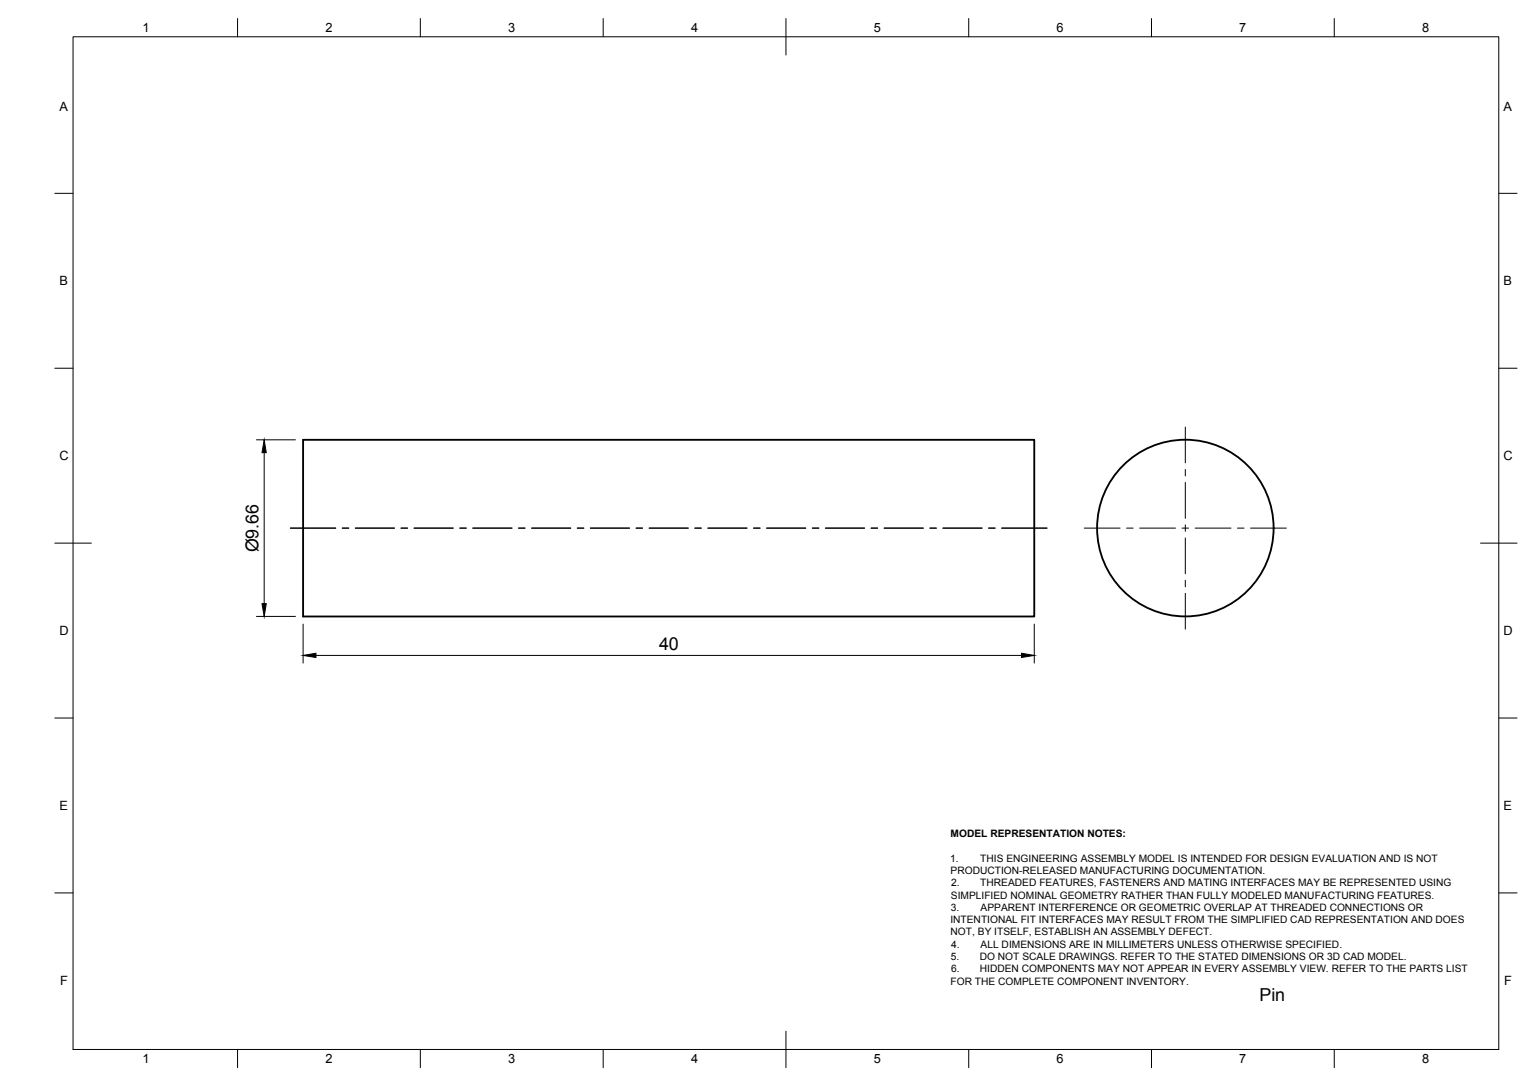
ISO-10303-21;
HEADER;
/* Generated by software containing ST-Developer
 * from STEP Tools, Inc. (www.steptools.com) 
 */

FILE_DESCRIPTION(
/* description */ ('STEP AP214'),
/* implementation_level */ '2;1');

FILE_NAME(
/* name */ 'PIN.step',
/* time_stamp */ '2026-10-06T11:20:11-07:00',
/* author */ (''),
/* organization */ (''),
/* preprocessor_version */ 'ST-DEVELOPER v20.2',
/* originating_system */ 'Autodesk Translation Framework v15.15.0.0',
/* authorisation */ '');

FILE_SCHEMA (('AUTOMOTIVE_DESIGN { 1 0 10303 214 3 1 1 }'));
ENDSEC;

DATA;
#10=MECHANICAL_DESIGN_GEOMETRIC_PRESENTATION_REPRESENTATION('',(#50),#2840);
#38=SHAPE_REPRESENTATION_RELATIONSHIP('SRR','None',#2869,#44);
#44=ADVANCED_BREP_SHAPE_REPRESENTATION('',(#56),#2837);
#50=STYLED_ITEM('',(#2905),#56);
#56=MANIFOLD_SOLID_BREP('Body1',#1550);
#109=PLANE('',#1747);
#110=PLANE('',#1748);
#175=FACE_OUTER_BOUND('',#290,.T.);
#176=FACE_OUTER_BOUND('',#291,.T.);
#177=FACE_OUTER_BOUND('',#292,.T.);
#290=EDGE_LOOP('',(#1202,#1203,#1204,#1205));
#291=EDGE_LOOP('',(#1206));
#292=EDGE_LOOP('',(#1207));
#373=LINE('',#2610,#466);
#466=VECTOR('',#2132,4.83000000000002);
#590=CIRCLE('',#1745,4.83000000000002);
#591=CIRCLE('',#1746,4.83000000000002);
#705=VERTEX_POINT('',#2607);
#706=VERTEX_POINT('',#2609);
#882=EDGE_CURVE('',#705,#705,#590,.T.);
#883=EDGE_CURVE('',#705,#706,#373,.T.);
#884=EDGE_CURVE('',#706,#706,#591,.T.);
#1202=ORIENTED_EDGE('',*,*,#882,.T.);
#1203=ORIENTED_EDGE('',*,*,#883,.T.);
#1204=ORIENTED_EDGE('',*,*,#884,.F.);
#1205=ORIENTED_EDGE('',*,*,#883,.F.);
#1206=ORIENTED_EDGE('',*,*,#884,.T.);
#1207=ORIENTED_EDGE('',*,*,#882,.F.);
#1433=CYLINDRICAL_SURFACE('',#1744,4.83000000000002);
#1506=ADVANCED_FACE('',(#175),#1433,.T.);
#1507=ADVANCED_FACE('',(#176),#109,.T.);
#1508=ADVANCED_FACE('',(#177),#110,.F.);
#1550=CLOSED_SHELL('',(#1506,#1507,#1508));
#1743=AXIS2_PLACEMENT_3D('',#2605,#2126,#2127);
#1744=AXIS2_PLACEMENT_3D('',#2606,#2128,#2129);
#1745=AXIS2_PLACEMENT_3D('',#2608,#2130,#2131);
#1746=AXIS2_PLACEMENT_3D('',#2611,#2133,#2134);
#1747=AXIS2_PLACEMENT_3D('',#2612,#2135,#2136);
#1748=AXIS2_PLACEMENT_3D('',#2613,#2137,#2138);
#2126=DIRECTION('axis',(0.,0.,1.));
#2127=DIRECTION('refdir',(1.,0.,0.));
#2128=DIRECTION('center_axis',(0.,-1.,0.));
#2129=DIRECTION('ref_axis',(-5.55111512312576E-17,0.,-1.));
#2130=DIRECTION('center_axis',(0.,1.,0.));
#2131=DIRECTION('ref_axis',(5.55111512312576E-17,0.,1.));
#2132=DIRECTION('',(0.,1.,0.));
#2133=DIRECTION('center_axis',(0.,1.,0.));
#2134=DIRECTION('ref_axis',(5.55111512312576E-17,0.,1.));
#2135=DIRECTION('center_axis',(0.,1.,0.));
#2136=DIRECTION('ref_axis',(5.55111512312576E-17,0.,1.));
#2137=DIRECTION('center_axis',(0.,1.,0.));
#2138=DIRECTION('ref_axis',(5.55111512312576E-17,0.,1.));
#2605=CARTESIAN_POINT('',(0.,0.,0.));
#2606=CARTESIAN_POINT('Origin',(0.,40.,0.));
#2607=CARTESIAN_POINT('',(-3.23385543541199E-16,0.,4.83000000000002));
#2608=CARTESIAN_POINT('Origin',(0.,0.,0.));
#2609=CARTESIAN_POINT('',(-3.23385543541199E-16,40.,4.83000000000002));
#2610=CARTESIAN_POINT('',(-3.23385543541199E-16,40.,4.83000000000002));
#2611=CARTESIAN_POINT('Origin',(0.,40.,0.));
#2612=CARTESIAN_POINT('Origin',(0.,40.,0.));
#2613=CARTESIAN_POINT('Origin',(0.,0.,0.));
#2829=UNCERTAINTY_MEASURE_WITH_UNIT(LENGTH_MEASURE(0.01),#2841,
'DISTANCE_ACCURACY_VALUE',
'Maximum model space distance between geometric entities at asserted c
onnectivities');
#2832=UNCERTAINTY_MEASURE_WITH_UNIT(LENGTH_MEASURE(0.01),#2841,
'DISTANCE_ACCURACY_VALUE',
'Maximum model space distance between geometric entities at asserted c
onnectivities');
#2837=(
GEOMETRIC_REPRESENTATION_CONTEXT(3)
GLOBAL_UNCERTAINTY_ASSIGNED_CONTEXT((#2829))
GLOBAL_UNIT_ASSIGNED_CONTEXT((#2841,#2843,#2844))
REPRESENTATION_CONTEXT('','3D')
);
#2840=(
GEOMETRIC_REPRESENTATION_CONTEXT(3)
GLOBAL_UNCERTAINTY_ASSIGNED_CONTEXT((#2832))
GLOBAL_UNIT_ASSIGNED_CONTEXT((#2841,#2843,#2844))
REPRESENTATION_CONTEXT('','3D')
);
#2841=(
LENGTH_UNIT()
NAMED_UNIT(*)
SI_UNIT(.MILLI.,.METRE.)
);
#2843=(
NAMED_UNIT(*)
PLANE_ANGLE_UNIT()
SI_UNIT($,.RADIAN.)
);
#2844=(
NAMED_UNIT(*)
SI_UNIT($,.STERADIAN.)
SOLID_ANGLE_UNIT()
);
#2849=SHAPE_DEFINITION_REPRESENTATION(#2856,#2869);
#2856=PRODUCT_DEFINITION_SHAPE('',$,#2877);
#2869=SHAPE_REPRESENTATION('',(#1743),#2837);
#2872=PRODUCT_DEFINITION_CONTEXT('part definition',#2895,'design');
#2877=PRODUCT_DEFINITION('Pin','PIN',#2884,#2872);
#2884=PRODUCT_DEFINITION_FORMATION('',$,#2901);
#2895=APPLICATION_CONTEXT(
'Core Data for Automotive Mechanical Design Process');
#2896=PRODUCT_CONTEXT('part definition',#2895,'mechanical');
#2901=PRODUCT('Pin','PIN',$,(#2896));
#2905=PRESENTATION_STYLE_ASSIGNMENT((#2907));
#2907=SURFACE_STYLE_USAGE(.BOTH.,#2909);
#2909=SURFACE_SIDE_STYLE('',(#2911));
#2911=SURFACE_STYLE_FILL_AREA(#2913);
#2913=FILL_AREA_STYLE('Opaque(202,209,238)',(#2915));
#2915=FILL_AREA_STYLE_COLOUR('Opaque(202,209,238)',#2917);
#2917=COLOUR_RGB('Opaque(202,209,238)', 0.66274510, 0.83137255, 0.94901961);
ENDSEC;
END-ISO-10303-21;
